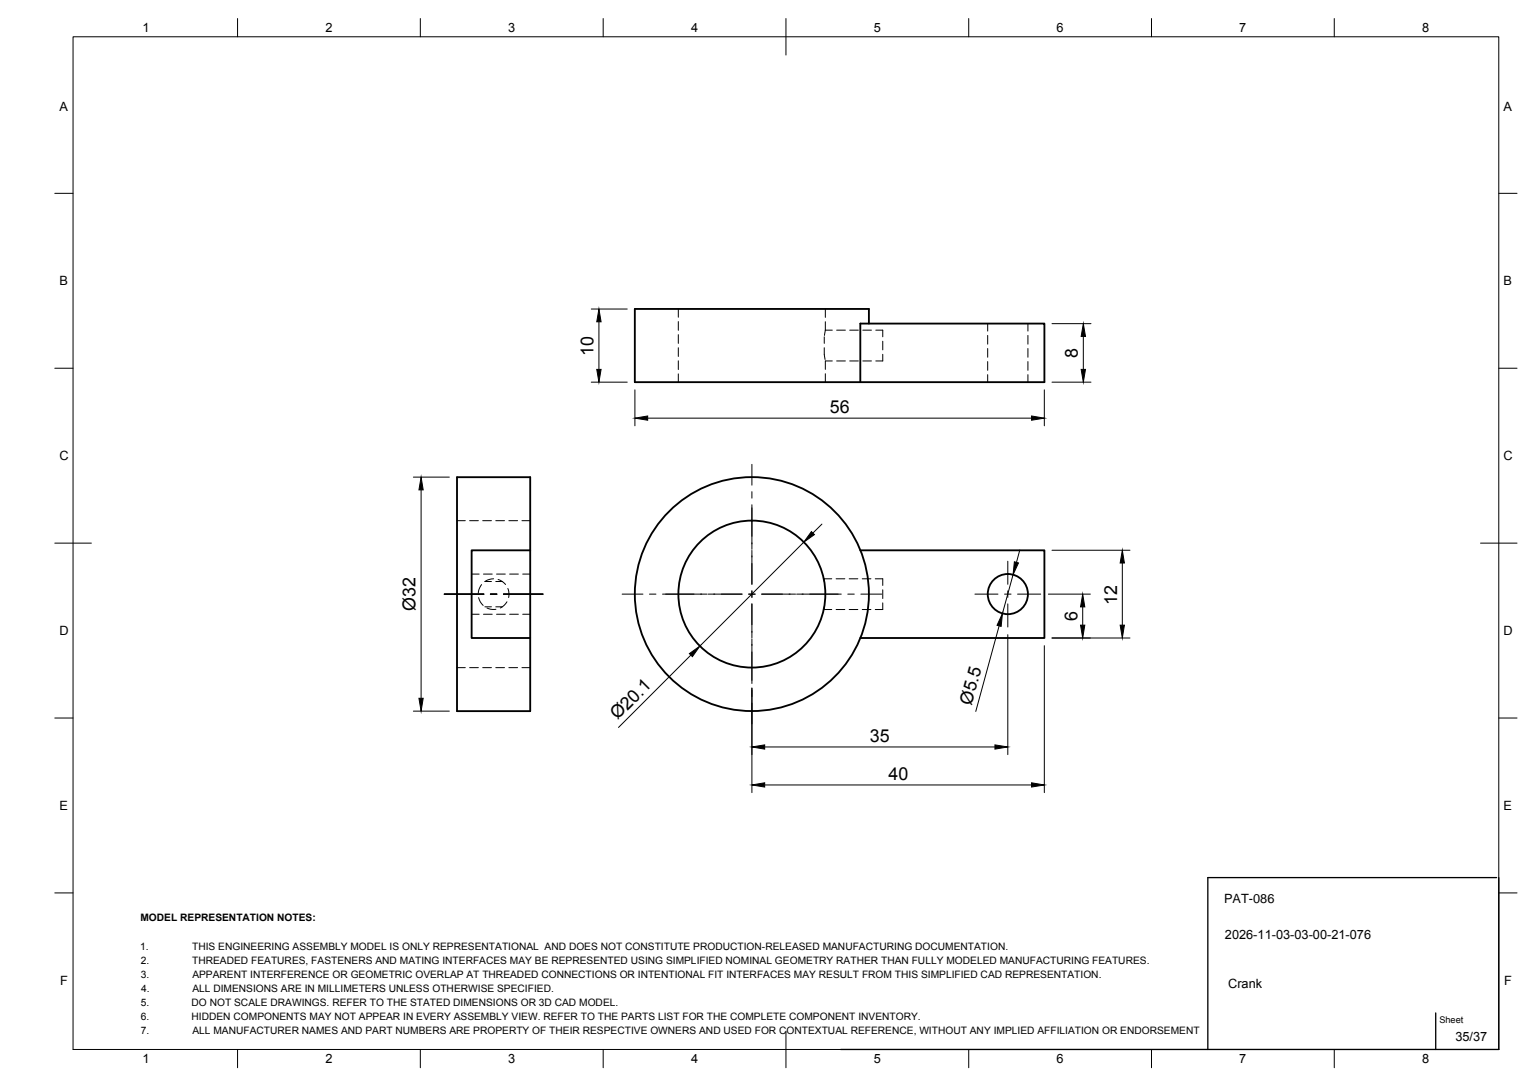
ISO-10303-21;
HEADER;
/* Generated by software containing ST-Developer
 * from STEP Tools, Inc. (www.steptools.com) 
 */

FILE_DESCRIPTION(
/* description */ ('Ratchet and pawl hand winch drum'),
/* implementation_level */ '2;1');

FILE_NAME(
/* name */ 'Crank.step',
/* time_stamp */ '2026-10-27T12:42:58-07:00',
/* author */ (''),
/* organization */ (''),
/* preprocessor_version */ 'ST-DEVELOPER v20.2',
/* originating_system */ 'Autodesk Translation Framework v15.17.0.0',
/* authorisation */ '');

FILE_SCHEMA (('AUTOMOTIVE_DESIGN { 1 0 10303 214 3 1 1 }'));
ENDSEC;

DATA;
#10=MECHANICAL_DESIGN_GEOMETRIC_PRESENTATION_REPRESENTATION('',(#419),#11801);
#317=B_SPLINE_CURVE_WITH_KNOTS('',3,(#11413,#11414,#11415,#11416,#11417,
#11418,#11419,#11420,#11421,#11422,#11423,#11424,#11425,#11426),
 .UNSPECIFIED.,.F.,.F.,(4,2,2,2,2,2,4),(0.75600573798702,0.793568827564648,
0.872922520054202,0.952276212543757,1.03162990503331,1.11098359752287,1.14854668710049),
 .UNSPECIFIED.);
#318=B_SPLINE_CURVE_WITH_KNOTS('',3,(#11434,#11435,#11436,#11437,#11438,
#11439,#11440,#11441,#11442,#11443,#11444,#11445,#11446,#11447),
 .UNSPECIFIED.,.F.,.F.,(4,2,2,2,2,2,4),(0.121154929624516,0.158718019202143,
0.238071711691698,0.317425404181252,0.396779096670807,0.476132789160362,
0.51369587873799),.UNSPECIFIED.);
#350=SHAPE_REPRESENTATION_RELATIONSHIP('SRR','None',#11978,#384);
#384=ADVANCED_BREP_SHAPE_REPRESENTATION('',(#452),#11795);
#419=STYLED_ITEM('',(#12227),#452);
#452=MANIFOLD_SOLID_BREP('Body1',#6298);
#591=FACE_BOUND('',#1639,.T.);
#592=FACE_BOUND('',#1640,.T.);
#593=FACE_BOUND('',#1643,.T.);
#594=FACE_BOUND('',#1648,.T.);
#595=FACE_BOUND('',#1650,.T.);
#803=PLANE('',#7211);
#804=PLANE('',#7217);
#805=PLANE('',#7218);
#806=PLANE('',#7219);
#807=PLANE('',#7223);
#808=PLANE('',#7224);
#809=PLANE('',#7226);
#810=PLANE('',#7227);
#811=PLANE('',#7232);
#1142=FACE_OUTER_BOUND('',#1633,.T.);
#1143=FACE_OUTER_BOUND('',#1634,.T.);
#1144=FACE_OUTER_BOUND('',#1635,.T.);
#1145=FACE_OUTER_BOUND('',#1636,.T.);
#1146=FACE_OUTER_BOUND('',#1637,.T.);
#1147=FACE_OUTER_BOUND('',#1638,.T.);
#1148=FACE_OUTER_BOUND('',#1641,.T.);
#1149=FACE_OUTER_BOUND('',#1642,.T.);
#1150=FACE_OUTER_BOUND('',#1644,.T.);
#1151=FACE_OUTER_BOUND('',#1645,.T.);
#1152=FACE_OUTER_BOUND('',#1646,.T.);
#1153=FACE_OUTER_BOUND('',#1647,.T.);
#1154=FACE_OUTER_BOUND('',#1649,.T.);
#1633=EDGE_LOOP('',(#5591,#5592,#5593,#5594));
#1634=EDGE_LOOP('',(#5595,#5596));
#1635=EDGE_LOOP('',(#5597,#5598,#5599,#5600,#5601,#5602,#5603,#5604));
#1636=EDGE_LOOP('',(#5605));
#1637=EDGE_LOOP('',(#5606,#5607,#5608));
#1638=EDGE_LOOP('',(#5609,#5610,#5611,#5612,#5613));
#1639=EDGE_LOOP('',(#5614));
#1640=EDGE_LOOP('',(#5615));
#1641=EDGE_LOOP('',(#5616,#5617,#5618,#5619));
#1642=EDGE_LOOP('',(#5620,#5621,#5622,#5623));
#1643=EDGE_LOOP('',(#5624));
#1644=EDGE_LOOP('',(#5625,#5626,#5627,#5628));
#1645=EDGE_LOOP('',(#5629,#5630,#5631,#5632));
#1646=EDGE_LOOP('',(#5633,#5634,#5635,#5636,#5637,#5638,#5639,#5640));
#1647=EDGE_LOOP('',(#5641,#5642,#5643,#5644));
#1648=EDGE_LOOP('',(#5645,#5646,#5647,#5648));
#1649=EDGE_LOOP('',(#5649));
#1650=EDGE_LOOP('',(#5650));
#2134=LINE('',#11404,#2645);
#2135=LINE('',#11409,#2646);
#2136=LINE('',#11430,#2647);
#2137=LINE('',#11450,#2648);
#2138=LINE('',#11456,#2649);
#2139=LINE('',#11458,#2650);
#2140=LINE('',#11460,#2651);
#2141=LINE('',#11466,#2652);
#2142=LINE('',#11468,#2653);
#2143=LINE('',#11469,#2654);
#2144=LINE('',#11474,#2655);
#2145=LINE('',#11475,#2656);
#2146=LINE('',#11477,#2657);
#2147=LINE('',#11478,#2658);
#2148=LINE('',#11483,#2659);
#2149=LINE('',#11487,#2660);
#2645=VECTOR('',#8857,0.275);
#2646=VECTOR('',#8862,1.);
#2647=VECTOR('',#8869,0.21);
#2648=VECTOR('',#8878,1.);
#2649=VECTOR('',#8883,1.);
#2650=VECTOR('',#8884,1.);
#2651=VECTOR('',#8885,1.);
#2652=VECTOR('',#8892,1.);
#2653=VECTOR('',#8893,1.);
#2654=VECTOR('',#8894,1.);
#2655=VECTOR('',#8899,1.);
#2656=VECTOR('',#8900,1.);
#2657=VECTOR('',#8903,1.);
#2658=VECTOR('',#8904,1.);
#2659=VECTOR('',#8911,1.6);
#2660=VECTOR('',#8916,1.005);
#2910=CIRCLE('',#7209,0.275);
#2911=CIRCLE('',#7210,0.275);
#2912=CIRCLE('',#7212,0.21);
#2913=CIRCLE('',#7214,0.21);
#2914=CIRCLE('',#7215,0.21);
#2915=CIRCLE('',#7216,0.21);
#2916=CIRCLE('',#7220,1.6);
#2917=CIRCLE('',#7221,1.6);
#2918=CIRCLE('',#7222,1.005);
#2919=CIRCLE('',#7225,1.6);
#2920=CIRCLE('',#7229,1.6);
#2921=CIRCLE('',#7231,1.005);
#3397=VERTEX_POINT('',#11401);
#3398=VERTEX_POINT('',#11403);
#3399=VERTEX_POINT('',#11407);
#3400=VERTEX_POINT('',#11408);
#3401=VERTEX_POINT('',#11412);
#3402=VERTEX_POINT('',#11427);
#3403=VERTEX_POINT('',#11429);
#3404=VERTEX_POINT('',#11432);
#3405=VERTEX_POINT('',#11452);
#3406=VERTEX_POINT('',#11453);
#3407=VERTEX_POINT('',#11455);
#3408=VERTEX_POINT('',#11457);
#3409=VERTEX_POINT('',#11459);
#3410=VERTEX_POINT('',#11462);
#3411=VERTEX_POINT('',#11465);
#3412=VERTEX_POINT('',#11467);
#3413=VERTEX_POINT('',#11471);
#3414=VERTEX_POINT('',#11473);
#3415=VERTEX_POINT('',#11481);
#3416=VERTEX_POINT('',#11485);
#4139=EDGE_CURVE('',#3397,#3397,#2910,.T.);
#4140=EDGE_CURVE('',#3397,#3398,#2134,.T.);
#4141=EDGE_CURVE('',#3398,#3398,#2911,.T.);
#4142=EDGE_CURVE('',#3399,#3400,#2135,.T.);
#4143=EDGE_CURVE('',#3399,#3400,#2912,.T.);
#4144=EDGE_CURVE('',#3401,#3399,#317,.T.);
#4145=EDGE_CURVE('',#3402,#3401,#2913,.T.);
#4146=EDGE_CURVE('',#3402,#3403,#2136,.T.);
#4147=EDGE_CURVE('',#3403,#3403,#2914,.T.);
#4148=EDGE_CURVE('',#3404,#3402,#2915,.T.);
#4149=EDGE_CURVE('',#3400,#3404,#318,.T.);
#4150=EDGE_CURVE('',#3404,#3401,#2137,.T.);
#4151=EDGE_CURVE('',#3405,#3406,#2916,.T.);
#4152=EDGE_CURVE('',#3405,#3407,#2138,.T.);
#4153=EDGE_CURVE('',#3407,#3408,#2139,.T.);
#4154=EDGE_CURVE('',#3408,#3409,#2140,.T.);
#4155=EDGE_CURVE('',#3406,#3409,#2917,.T.);
#4156=EDGE_CURVE('',#3410,#3410,#2918,.T.);
#4157=EDGE_CURVE('',#3409,#3411,#2141,.T.);
#4158=EDGE_CURVE('',#3408,#3412,#2142,.T.);
#4159=EDGE_CURVE('',#3411,#3412,#2143,.T.);
#4160=EDGE_CURVE('',#3411,#3413,#2919,.T.);
#4161=EDGE_CURVE('',#3412,#3414,#2144,.T.);
#4162=EDGE_CURVE('',#3414,#3413,#2145,.T.);
#4163=EDGE_CURVE('',#3413,#3405,#2146,.T.);
#4164=EDGE_CURVE('',#3407,#3414,#2147,.T.);
#4165=EDGE_CURVE('',#3415,#3415,#2920,.T.);
#4166=EDGE_CURVE('',#3415,#3406,#2148,.T.);
#4167=EDGE_CURVE('',#3416,#3416,#2921,.T.);
#4168=EDGE_CURVE('',#3416,#3410,#2149,.T.);
#5591=ORIENTED_EDGE('',*,*,#4139,.F.);
#5592=ORIENTED_EDGE('',*,*,#4140,.T.);
#5593=ORIENTED_EDGE('',*,*,#4141,.F.);
#5594=ORIENTED_EDGE('',*,*,#4140,.F.);
#5595=ORIENTED_EDGE('',*,*,#4142,.F.);
#5596=ORIENTED_EDGE('',*,*,#4143,.T.);
#5597=ORIENTED_EDGE('',*,*,#4144,.F.);
#5598=ORIENTED_EDGE('',*,*,#4145,.F.);
#5599=ORIENTED_EDGE('',*,*,#4146,.T.);
#5600=ORIENTED_EDGE('',*,*,#4147,.T.);
#5601=ORIENTED_EDGE('',*,*,#4146,.F.);
#5602=ORIENTED_EDGE('',*,*,#4148,.F.);
#5603=ORIENTED_EDGE('',*,*,#4149,.F.);
#5604=ORIENTED_EDGE('',*,*,#4143,.F.);
#5605=ORIENTED_EDGE('',*,*,#4147,.F.);
#5606=ORIENTED_EDGE('',*,*,#4150,.F.);
#5607=ORIENTED_EDGE('',*,*,#4148,.T.);
#5608=ORIENTED_EDGE('',*,*,#4145,.T.);
#5609=ORIENTED_EDGE('',*,*,#4151,.F.);
#5610=ORIENTED_EDGE('',*,*,#4152,.T.);
#5611=ORIENTED_EDGE('',*,*,#4153,.T.);
#5612=ORIENTED_EDGE('',*,*,#4154,.T.);
#5613=ORIENTED_EDGE('',*,*,#4155,.F.);
#5614=ORIENTED_EDGE('',*,*,#4139,.T.);
#5615=ORIENTED_EDGE('',*,*,#4156,.F.);
#5616=ORIENTED_EDGE('',*,*,#4157,.F.);
#5617=ORIENTED_EDGE('',*,*,#4154,.F.);
#5618=ORIENTED_EDGE('',*,*,#4158,.T.);
#5619=ORIENTED_EDGE('',*,*,#4159,.F.);
#5620=ORIENTED_EDGE('',*,*,#4160,.F.);
#5621=ORIENTED_EDGE('',*,*,#4159,.T.);
#5622=ORIENTED_EDGE('',*,*,#4161,.T.);
#5623=ORIENTED_EDGE('',*,*,#4162,.T.);
#5624=ORIENTED_EDGE('',*,*,#4141,.T.);
#5625=ORIENTED_EDGE('',*,*,#4163,.F.);
#5626=ORIENTED_EDGE('',*,*,#4162,.F.);
#5627=ORIENTED_EDGE('',*,*,#4164,.F.);
#5628=ORIENTED_EDGE('',*,*,#4152,.F.);
#5629=ORIENTED_EDGE('',*,*,#4153,.F.);
#5630=ORIENTED_EDGE('',*,*,#4164,.T.);
#5631=ORIENTED_EDGE('',*,*,#4161,.F.);
#5632=ORIENTED_EDGE('',*,*,#4158,.F.);
#5633=ORIENTED_EDGE('',*,*,#4165,.F.);
#5634=ORIENTED_EDGE('',*,*,#4166,.T.);
#5635=ORIENTED_EDGE('',*,*,#4155,.T.);
#5636=ORIENTED_EDGE('',*,*,#4157,.T.);
#5637=ORIENTED_EDGE('',*,*,#4160,.T.);
#5638=ORIENTED_EDGE('',*,*,#4163,.T.);
#5639=ORIENTED_EDGE('',*,*,#4151,.T.);
#5640=ORIENTED_EDGE('',*,*,#4166,.F.);
#5641=ORIENTED_EDGE('',*,*,#4167,.F.);
#5642=ORIENTED_EDGE('',*,*,#4168,.T.);
#5643=ORIENTED_EDGE('',*,*,#4156,.T.);
#5644=ORIENTED_EDGE('',*,*,#4168,.F.);
#5645=ORIENTED_EDGE('',*,*,#4149,.T.);
#5646=ORIENTED_EDGE('',*,*,#4150,.T.);
#5647=ORIENTED_EDGE('',*,*,#4144,.T.);
#5648=ORIENTED_EDGE('',*,*,#4142,.T.);
#5649=ORIENTED_EDGE('',*,*,#4165,.T.);
#5650=ORIENTED_EDGE('',*,*,#4167,.T.);
#5899=CYLINDRICAL_SURFACE('',#7208,0.275);
#5900=CYLINDRICAL_SURFACE('',#7213,0.21);
#5901=CYLINDRICAL_SURFACE('',#7228,1.6);
#5902=CYLINDRICAL_SURFACE('',#7230,1.005);
#6212=ADVANCED_FACE('',(#1142),#5899,.F.);
#6213=ADVANCED_FACE('',(#1143),#803,.T.);
#6214=ADVANCED_FACE('',(#1144),#5900,.F.);
#6215=ADVANCED_FACE('',(#1145),#804,.F.);
#6216=ADVANCED_FACE('',(#1146),#805,.T.);
#6217=ADVANCED_FACE('',(#1147,#591,#592),#806,.F.);
#6218=ADVANCED_FACE('',(#1148),#807,.T.);
#6219=ADVANCED_FACE('',(#1149,#593),#808,.T.);
#6220=ADVANCED_FACE('',(#1150),#809,.T.);
#6221=ADVANCED_FACE('',(#1151),#810,.T.);
#6222=ADVANCED_FACE('',(#1152),#5901,.T.);
#6223=ADVANCED_FACE('',(#1153,#594),#5902,.F.);
#6224=ADVANCED_FACE('',(#1154,#595),#811,.T.);
#6298=CLOSED_SHELL('',(#6212,#6213,#6214,#6215,#6216,#6217,#6218,#6219,
#6220,#6221,#6222,#6223,#6224));
#7207=AXIS2_PLACEMENT_3D('',#11399,#8851,#8852);
#7208=AXIS2_PLACEMENT_3D('',#11400,#8853,#8854);
#7209=AXIS2_PLACEMENT_3D('',#11402,#8855,#8856);
#7210=AXIS2_PLACEMENT_3D('',#11405,#8858,#8859);
#7211=AXIS2_PLACEMENT_3D('',#11406,#8860,#8861);
#7212=AXIS2_PLACEMENT_3D('',#11410,#8863,#8864);
#7213=AXIS2_PLACEMENT_3D('',#11411,#8865,#8866);
#7214=AXIS2_PLACEMENT_3D('',#11428,#8867,#8868);
#7215=AXIS2_PLACEMENT_3D('',#11431,#8870,#8871);
#7216=AXIS2_PLACEMENT_3D('',#11433,#8872,#8873);
#7217=AXIS2_PLACEMENT_3D('',#11448,#8874,#8875);
#7218=AXIS2_PLACEMENT_3D('',#11449,#8876,#8877);
#7219=AXIS2_PLACEMENT_3D('',#11451,#8879,#8880);
#7220=AXIS2_PLACEMENT_3D('',#11454,#8881,#8882);
#7221=AXIS2_PLACEMENT_3D('',#11461,#8886,#8887);
#7222=AXIS2_PLACEMENT_3D('',#11463,#8888,#8889);
#7223=AXIS2_PLACEMENT_3D('',#11464,#8890,#8891);
#7224=AXIS2_PLACEMENT_3D('',#11470,#8895,#8896);
#7225=AXIS2_PLACEMENT_3D('',#11472,#8897,#8898);
#7226=AXIS2_PLACEMENT_3D('',#11476,#8901,#8902);
#7227=AXIS2_PLACEMENT_3D('',#11479,#8905,#8906);
#7228=AXIS2_PLACEMENT_3D('',#11480,#8907,#8908);
#7229=AXIS2_PLACEMENT_3D('',#11482,#8909,#8910);
#7230=AXIS2_PLACEMENT_3D('',#11484,#8912,#8913);
#7231=AXIS2_PLACEMENT_3D('',#11486,#8914,#8915);
#7232=AXIS2_PLACEMENT_3D('',#11488,#8917,#8918);
#8851=DIRECTION('axis',(0.,0.,1.));
#8852=DIRECTION('refdir',(1.,0.,0.));
#8853=DIRECTION('center_axis',(0.,1.,0.));
#8854=DIRECTION('ref_axis',(1.,0.,0.));
#8855=DIRECTION('center_axis',(0.,1.,0.));
#8856=DIRECTION('ref_axis',(1.,0.,0.));
#8857=DIRECTION('',(0.,1.,0.));
#8858=DIRECTION('center_axis',(0.,-1.,0.));
#8859=DIRECTION('ref_axis',(1.,0.,0.));
#8860=DIRECTION('center_axis',(0.,0.,1.));
#8861=DIRECTION('ref_axis',(1.,0.,0.));
#8862=DIRECTION('',(0.,1.,0.));
#8863=DIRECTION('center_axis',(0.,0.,1.));
#8864=DIRECTION('ref_axis',(1.,0.,0.));
#8865=DIRECTION('center_axis',(0.,0.,1.));
#8866=DIRECTION('ref_axis',(1.,0.,0.));
#8867=DIRECTION('center_axis',(0.,0.,1.));
#8868=DIRECTION('ref_axis',(1.,0.,0.));
#8869=DIRECTION('',(0.,0.,1.));
#8870=DIRECTION('center_axis',(0.,0.,1.));
#8871=DIRECTION('ref_axis',(1.,0.,0.));
#8872=DIRECTION('center_axis',(0.,0.,1.));
#8873=DIRECTION('ref_axis',(1.,0.,0.));
#8874=DIRECTION('center_axis',(0.,0.,1.));
#8875=DIRECTION('ref_axis',(1.,0.,0.));
#8876=DIRECTION('center_axis',(0.,0.,1.));
#8877=DIRECTION('ref_axis',(1.,0.,0.));
#8878=DIRECTION('',(0.,-1.,0.));
#8879=DIRECTION('center_axis',(0.,1.,0.));
#8880=DIRECTION('ref_axis',(1.,0.,0.));
#8881=DIRECTION('center_axis',(0.,1.,0.));
#8882=DIRECTION('ref_axis',(1.,0.,0.));
#8883=DIRECTION('',(0.,0.,1.));
#8884=DIRECTION('',(-1.,0.,0.));
#8885=DIRECTION('',(0.,0.,-1.));
#8886=DIRECTION('center_axis',(0.,1.,0.));
#8887=DIRECTION('ref_axis',(1.,0.,0.));
#8888=DIRECTION('center_axis',(0.,-1.,0.));
#8889=DIRECTION('ref_axis',(1.,0.,0.));
#8890=DIRECTION('center_axis',(-1.,0.,0.));
#8891=DIRECTION('ref_axis',(0.,0.,1.));
#8892=DIRECTION('',(0.,1.,0.));
#8893=DIRECTION('',(0.,1.,0.));
#8894=DIRECTION('',(0.,0.,1.));
#8895=DIRECTION('center_axis',(0.,1.,0.));
#8896=DIRECTION('ref_axis',(0.,0.,1.));
#8897=DIRECTION('center_axis',(0.,1.,0.));
#8898=DIRECTION('ref_axis',(1.,0.,0.));
#8899=DIRECTION('',(1.,0.,0.));
#8900=DIRECTION('',(0.,0.,-1.));
#8901=DIRECTION('center_axis',(1.,0.,0.));
#8902=DIRECTION('ref_axis',(0.,0.,-1.));
#8903=DIRECTION('',(0.,-1.,0.));
#8904=DIRECTION('',(0.,1.,0.));
#8905=DIRECTION('center_axis',(0.,0.,1.));
#8906=DIRECTION('ref_axis',(1.,0.,0.));
#8907=DIRECTION('center_axis',(0.,1.,0.));
#8908=DIRECTION('ref_axis',(1.,0.,0.));
#8909=DIRECTION('center_axis',(0.,1.,0.));
#8910=DIRECTION('ref_axis',(1.,0.,0.));
#8911=DIRECTION('',(0.,-1.,0.));
#8912=DIRECTION('center_axis',(0.,1.,0.));
#8913=DIRECTION('ref_axis',(1.,0.,0.));
#8914=DIRECTION('center_axis',(0.,-1.,0.));
#8915=DIRECTION('ref_axis',(1.,0.,0.));
#8916=DIRECTION('',(0.,-1.,0.));
#8917=DIRECTION('center_axis',(0.,1.,0.));
#8918=DIRECTION('ref_axis',(1.,0.,0.));
#11399=CARTESIAN_POINT('',(0.,0.,0.));
#11400=CARTESIAN_POINT('Origin',(0.,-6.6,10.03));
#11401=CARTESIAN_POINT('',(-0.275,-6.5,10.03));
#11402=CARTESIAN_POINT('Origin',(0.,-6.5,10.03));
#11403=CARTESIAN_POINT('',(-0.275,-5.7,10.03));
#11404=CARTESIAN_POINT('',(-0.275,-6.6,10.03));
#11405=CARTESIAN_POINT('Origin',(0.,-5.7,10.03));
#11406=CARTESIAN_POINT('Origin',(0.,-6.,7.52));
#11407=CARTESIAN_POINT('',(0.172988438920056,-6.11905880899792,7.52));
#11408=CARTESIAN_POINT('',(0.172988438920056,-5.88094119100209,7.52));
#11409=CARTESIAN_POINT('',(0.172988438920056,-6.5,7.52));
#11410=CARTESIAN_POINT('Origin',(0.,-6.,7.52));
#11411=CARTESIAN_POINT('Origin',(0.,-6.,7.52));
#11412=CARTESIAN_POINT('',(-0.172988438920056,-6.11905880899792,7.52));
#11413=CARTESIAN_POINT('Ctrl Pts',(-0.172988438920056,-6.11905880899792,
7.52));
#11414=CARTESIAN_POINT('Ctrl Pts',(-0.165594865311313,-6.12980142239529,
7.52129192197638));
#11415=CARTESIAN_POINT('Ctrl Pts',(-0.157297138725606,-6.13968770937274,
7.52265394943905));
#11416=CARTESIAN_POINT('Ctrl Pts',(-0.129892073845076,-6.16709277425327,
7.5267480843909));
#11417=CARTESIAN_POINT('Ctrl Pts',(-0.106330167759284,-6.18324205633295,
7.52969589327638));
#11418=CARTESIAN_POINT('Ctrl Pts',(-0.05461290463241,-6.20469779396491,
7.53385029472357));
#11419=CARTESIAN_POINT('Ctrl Pts',(-0.0264512308298516,-6.21,7.535));
#11420=CARTESIAN_POINT('Ctrl Pts',(0.0264512308298515,-6.21,7.535));
#11421=CARTESIAN_POINT('Ctrl Pts',(0.0546129046324099,-6.20469779396491,
7.53385029472357));
#11422=CARTESIAN_POINT('Ctrl Pts',(0.106330167759284,-6.18324205633295,
7.52969589327638));
#11423=CARTESIAN_POINT('Ctrl Pts',(0.129892073845076,-6.16709277425327,
7.5267480843909));
#11424=CARTESIAN_POINT('Ctrl Pts',(0.157297138725606,-6.13968770937274,
7.52265394943905));
#11425=CARTESIAN_POINT('Ctrl Pts',(0.165594865311314,-6.12980142239529,
7.52129192197638));
#11426=CARTESIAN_POINT('Ctrl Pts',(0.172988438920056,-6.11905880899792,
7.52));
#11427=CARTESIAN_POINT('',(-0.21,-6.,7.52));
#11428=CARTESIAN_POINT('Origin',(0.,-6.,7.52));
#11429=CARTESIAN_POINT('',(-0.21,-6.,8.32));
#11430=CARTESIAN_POINT('',(-0.21,-6.,7.52));
#11431=CARTESIAN_POINT('Origin',(0.,-6.,8.32));
#11432=CARTESIAN_POINT('',(-0.172988438920056,-5.88094119100209,7.52));
#11433=CARTESIAN_POINT('Origin',(0.,-6.,7.52));
#11434=CARTESIAN_POINT('Ctrl Pts',(0.172988438920056,-5.88094119100209,
7.52));
#11435=CARTESIAN_POINT('Ctrl Pts',(0.165594865311314,-5.87019857760471,
7.52129192197638));
#11436=CARTESIAN_POINT('Ctrl Pts',(0.157297138725606,-5.86031229062726,
7.52265394943905));
#11437=CARTESIAN_POINT('Ctrl Pts',(0.129892073845076,-5.83290722574673,
7.5267480843909));
#11438=CARTESIAN_POINT('Ctrl Pts',(0.106330167759284,-5.81675794366705,
7.52969589327638));
#11439=CARTESIAN_POINT('Ctrl Pts',(0.05461290463241,-5.79530220603509,7.53385029472357));
#11440=CARTESIAN_POINT('Ctrl Pts',(0.0264512308298516,-5.79,7.535));
#11441=CARTESIAN_POINT('Ctrl Pts',(-0.0264512308298515,-5.79,7.535));
#11442=CARTESIAN_POINT('Ctrl Pts',(-0.0546129046324109,-5.79530220603509,
7.53385029472357));
#11443=CARTESIAN_POINT('Ctrl Pts',(-0.106330167759285,-5.81675794366705,
7.52969589327638));
#11444=CARTESIAN_POINT('Ctrl Pts',(-0.129892073845076,-5.83290722574673,
7.5267480843909));
#11445=CARTESIAN_POINT('Ctrl Pts',(-0.157297138725607,-5.86031229062726,
7.52265394943905));
#11446=CARTESIAN_POINT('Ctrl Pts',(-0.165594865311314,-5.87019857760471,
7.52129192197638));
#11447=CARTESIAN_POINT('Ctrl Pts',(-0.172988438920057,-5.88094119100209,
7.52));
#11448=CARTESIAN_POINT('Origin',(0.,-6.,8.32));
#11449=CARTESIAN_POINT('Origin',(0.,-6.,7.52));
#11450=CARTESIAN_POINT('',(-0.172988438920056,-6.5,7.52));
#11451=CARTESIAN_POINT('Origin',(0.,-6.5,6.53));
#11452=CARTESIAN_POINT('',(0.6,-6.5,8.01323969741913));
#11453=CARTESIAN_POINT('',(-1.6,-6.5,6.53));
#11454=CARTESIAN_POINT('Origin',(0.,-6.5,6.53));
#11455=CARTESIAN_POINT('',(0.6,-6.5,10.53));
#11456=CARTESIAN_POINT('',(0.6,-6.5,6.53));
#11457=CARTESIAN_POINT('',(-0.6,-6.5,10.53));
#11458=CARTESIAN_POINT('',(0.6,-6.5,10.53));
#11459=CARTESIAN_POINT('',(-0.6,-6.5,8.01323969741913));
#11460=CARTESIAN_POINT('',(-0.6,-6.5,10.53));
#11461=CARTESIAN_POINT('Origin',(0.,-6.5,6.53));
#11462=CARTESIAN_POINT('',(-1.005,-6.5,6.53));
#11463=CARTESIAN_POINT('Origin',(0.,-6.5,6.53));
#11464=CARTESIAN_POINT('Origin',(-0.6,-6.5,6.53));
#11465=CARTESIAN_POINT('',(-0.6,-5.7,8.01323969741913));
#11466=CARTESIAN_POINT('',(-0.6,-6.5,8.01323969741913));
#11467=CARTESIAN_POINT('',(-0.6,-5.7,10.53));
#11468=CARTESIAN_POINT('',(-0.6,-6.5,10.53));
#11469=CARTESIAN_POINT('',(-0.6,-5.7,10.53));
#11470=CARTESIAN_POINT('Origin',(0.,-5.7,8.53));
#11471=CARTESIAN_POINT('',(0.6,-5.7,8.01323969741913));
#11472=CARTESIAN_POINT('Origin',(0.,-5.7,6.53));
#11473=CARTESIAN_POINT('',(0.6,-5.7,10.53));
#11474=CARTESIAN_POINT('',(0.6,-5.7,10.53));
#11475=CARTESIAN_POINT('',(0.6,-5.7,6.53));
#11476=CARTESIAN_POINT('Origin',(0.6,-6.5,10.53));
#11477=CARTESIAN_POINT('',(0.6,-6.5,8.01323969741913));
#11478=CARTESIAN_POINT('',(0.6,-6.5,10.53));
#11479=CARTESIAN_POINT('Origin',(-0.6,-6.5,10.53));
#11480=CARTESIAN_POINT('Origin',(0.,-6.5,6.53));
#11481=CARTESIAN_POINT('',(-1.6,-5.5,6.53));
#11482=CARTESIAN_POINT('Origin',(0.,-5.5,6.53));
#11483=CARTESIAN_POINT('',(-1.6,-6.5,6.53));
#11484=CARTESIAN_POINT('Origin',(0.,-6.5,6.53));
#11485=CARTESIAN_POINT('',(-1.005,-5.5,6.53));
#11486=CARTESIAN_POINT('Origin',(0.,-5.5,6.53));
#11487=CARTESIAN_POINT('',(-1.005,-6.5,6.53));
#11488=CARTESIAN_POINT('Origin',(0.,-5.5,6.53));
#11755=UNCERTAINTY_MEASURE_WITH_UNIT(LENGTH_MEASURE(0.001),#11802,
'DISTANCE_ACCURACY_VALUE',
'Maximum model space distance between geometric entities at asserted c
onnectivities');
#11761=UNCERTAINTY_MEASURE_WITH_UNIT(LENGTH_MEASURE(0.001),#11802,
'DISTANCE_ACCURACY_VALUE',
'Maximum model space distance between geometric entities at asserted c
onnectivities');
#11795=(
GEOMETRIC_REPRESENTATION_CONTEXT(3)
GLOBAL_UNCERTAINTY_ASSIGNED_CONTEXT((#11755))
GLOBAL_UNIT_ASSIGNED_CONTEXT((#11802,#11804,#11805))
REPRESENTATION_CONTEXT('','3D')
);
#11801=(
GEOMETRIC_REPRESENTATION_CONTEXT(3)
GLOBAL_UNCERTAINTY_ASSIGNED_CONTEXT((#11761))
GLOBAL_UNIT_ASSIGNED_CONTEXT((#11802,#11804,#11805))
REPRESENTATION_CONTEXT('','3D')
);
#11802=(
LENGTH_UNIT()
NAMED_UNIT(*)
SI_UNIT(.CENTI.,.METRE.)
);
#11804=(
NAMED_UNIT(*)
PLANE_ANGLE_UNIT()
SI_UNIT($,.RADIAN.)
);
#11805=(
NAMED_UNIT(*)
SI_UNIT($,.STERADIAN.)
SOLID_ANGLE_UNIT()
);
#11839=SHAPE_DEFINITION_REPRESENTATION(#11880,#11978);
#11880=PRODUCT_DEFINITION_SHAPE('',$,#12018);
#11978=SHAPE_REPRESENTATION('',(#7207),#11795);
#11984=PRODUCT_DEFINITION_CONTEXT('part definition',#12103,'design');
#12018=PRODUCT_DEFINITION('Crank','Crank',#12057,#11984);
#12057=PRODUCT_DEFINITION_FORMATION('',$,#12138);
#12103=APPLICATION_CONTEXT(
'Core Data for Automotive Mechanical Design Process');
#12104=PRODUCT_CONTEXT('part definition',#12103,'mechanical');
#12138=PRODUCT('Crank','Crank','Crank',(#12104));
#12221=COLOUR_RGB('Off White',0.89,0.88,0.83);
#12222=FILL_AREA_STYLE_COLOUR('',#12221);
#12223=FILL_AREA_STYLE('',(#12222));
#12224=SURFACE_STYLE_FILL_AREA(#12223);
#12225=SURFACE_SIDE_STYLE('',(#12224));
#12226=SURFACE_STYLE_USAGE(.BOTH.,#12225);
#12227=PRESENTATION_STYLE_ASSIGNMENT((#12226));
ENDSEC;
END-ISO-10303-21;
